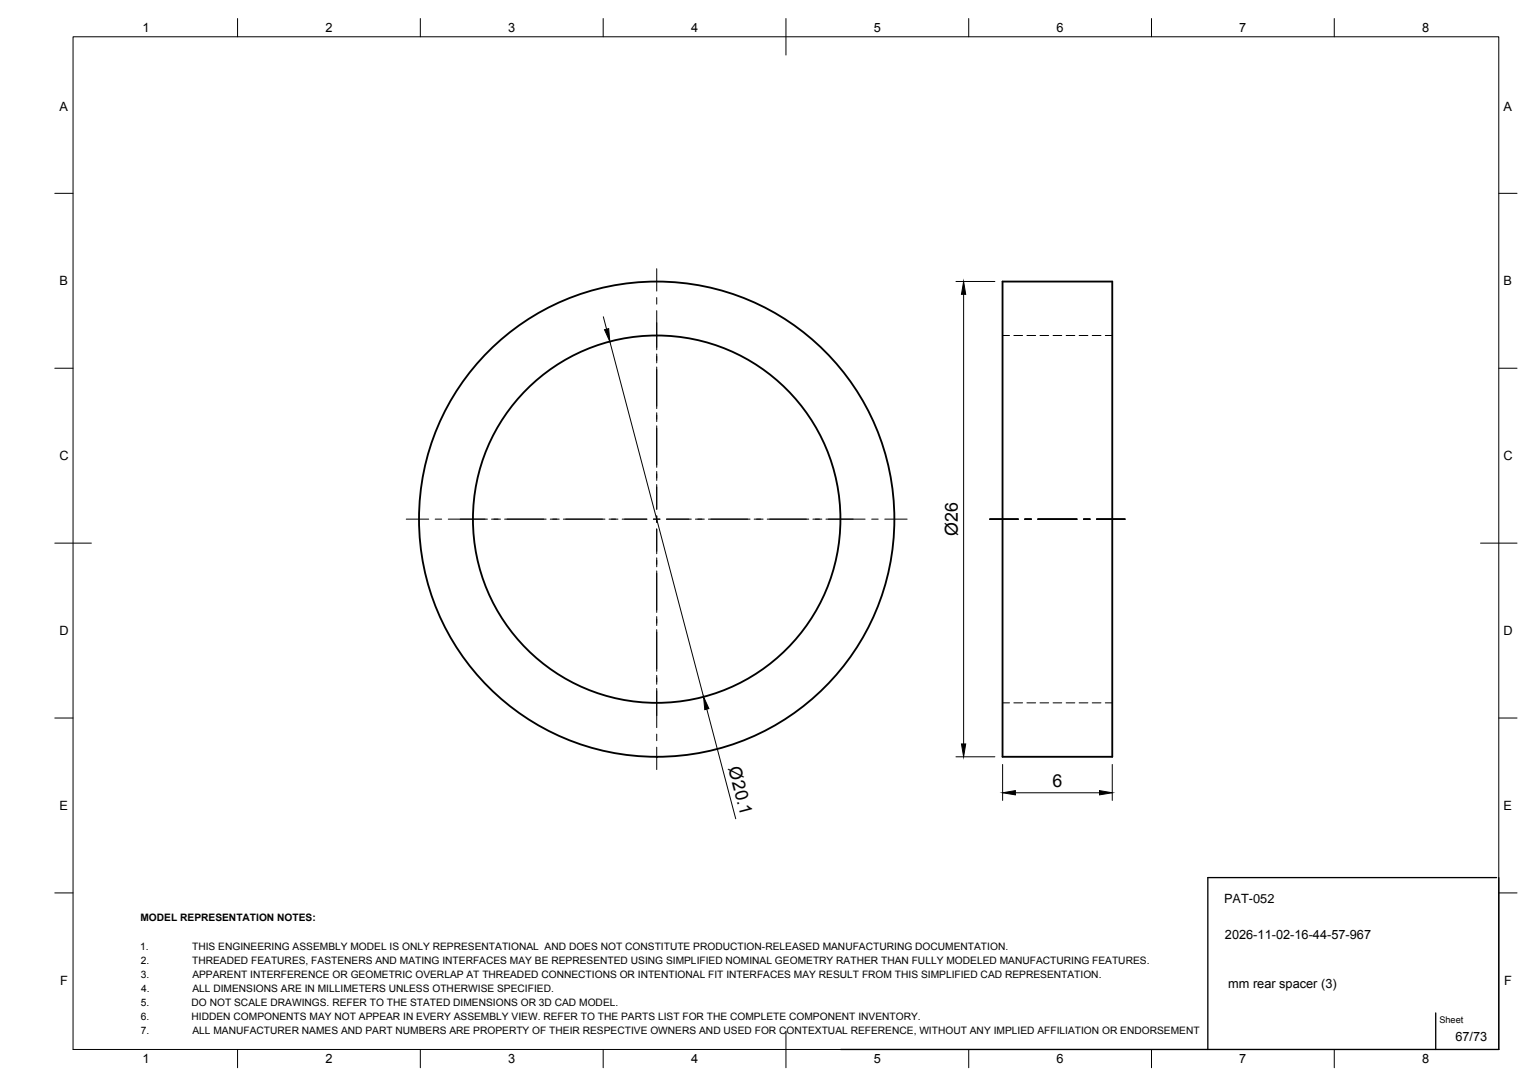
ISO-10303-21;
HEADER;
/* Generated by software containing ST-Developer
 * from STEP Tools, Inc. (www.steptools.com) 
 */

FILE_DESCRIPTION(
/* description */ ('Hand-crank gear train demonstrator'),
/* implementation_level */ '2;1');

FILE_NAME(
/* name */ 'mm rear spacer (3).step',
/* time_stamp */ '2026-10-28T03:22:13-07:00',
/* author */ (''),
/* organization */ (''),
/* preprocessor_version */ 'ST-DEVELOPER v20.2',
/* originating_system */ 'Autodesk Translation Framework v15.17.0.0',
/* authorisation */ '');

FILE_SCHEMA (('AUTOMOTIVE_DESIGN { 1 0 10303 214 3 1 1 }'));
ENDSEC;

DATA;
#10=MECHANICAL_DESIGN_GEOMETRIC_PRESENTATION_REPRESENTATION('',(#1257),#62758);
#1114=SHAPE_REPRESENTATION_RELATIONSHIP('SRR','None',#63092,#1178);
#1178=ADVANCED_BREP_SHAPE_REPRESENTATION('',(#1332),#62746);
#1257=STYLED_ITEM('',(#63476),#1332);
#1332=MANIFOLD_SOLID_BREP('Body1',#16441);
#1609=FACE_BOUND('',#4020,.T.);
#1610=FACE_BOUND('',#4022,.T.);
#2025=PLANE('',#18417);
#2026=PLANE('',#18418);
#2814=FACE_OUTER_BOUND('',#4017,.T.);
#2815=FACE_OUTER_BOUND('',#4018,.T.);
#2816=FACE_OUTER_BOUND('',#4019,.T.);
#2817=FACE_OUTER_BOUND('',#4021,.T.);
#4017=EDGE_LOOP('',(#13873,#13874,#13875,#13876));
#4018=EDGE_LOOP('',(#13877,#13878,#13879,#13880));
#4019=EDGE_LOOP('',(#13881));
#4020=EDGE_LOOP('',(#13882));
#4021=EDGE_LOOP('',(#13883));
#4022=EDGE_LOOP('',(#13884));
#5151=LINE('',#38498,#6283);
#5152=LINE('',#38504,#6284);
#6283=VECTOR('',#22206,1.005);
#6284=VECTOR('',#22213,1.3);
#7080=CIRCLE('',#18412,1.005);
#7081=CIRCLE('',#18413,1.005);
#7082=CIRCLE('',#18415,1.3);
#7083=CIRCLE('',#18416,1.3);
#8239=VERTEX_POINT('',#38495);
#8240=VERTEX_POINT('',#38497);
#8241=VERTEX_POINT('',#38501);
#8242=VERTEX_POINT('',#38503);
#10188=EDGE_CURVE('',#8239,#8239,#7080,.T.);
#10189=EDGE_CURVE('',#8239,#8240,#5151,.T.);
#10190=EDGE_CURVE('',#8240,#8240,#7081,.T.);
#10191=EDGE_CURVE('',#8241,#8241,#7082,.T.);
#10192=EDGE_CURVE('',#8241,#8242,#5152,.T.);
#10193=EDGE_CURVE('',#8242,#8242,#7083,.T.);
#13873=ORIENTED_EDGE('',*,*,#10188,.F.);
#13874=ORIENTED_EDGE('',*,*,#10189,.T.);
#13875=ORIENTED_EDGE('',*,*,#10190,.T.);
#13876=ORIENTED_EDGE('',*,*,#10189,.F.);
#13877=ORIENTED_EDGE('',*,*,#10191,.F.);
#13878=ORIENTED_EDGE('',*,*,#10192,.T.);
#13879=ORIENTED_EDGE('',*,*,#10193,.T.);
#13880=ORIENTED_EDGE('',*,*,#10192,.F.);
#13881=ORIENTED_EDGE('',*,*,#10191,.T.);
#13882=ORIENTED_EDGE('',*,*,#10188,.T.);
#13883=ORIENTED_EDGE('',*,*,#10193,.F.);
#13884=ORIENTED_EDGE('',*,*,#10190,.F.);
#15372=CYLINDRICAL_SURFACE('',#18411,1.005);
#15373=CYLINDRICAL_SURFACE('',#18414,1.3);
#16124=ADVANCED_FACE('',(#2814),#15372,.F.);
#16125=ADVANCED_FACE('',(#2815),#15373,.T.);
#16126=ADVANCED_FACE('',(#2816,#1609),#2025,.T.);
#16127=ADVANCED_FACE('',(#2817,#1610),#2026,.F.);
#16441=CLOSED_SHELL('',(#16124,#16125,#16126,#16127));
#18410=AXIS2_PLACEMENT_3D('',#38493,#22200,#22201);
#18411=AXIS2_PLACEMENT_3D('',#38494,#22202,#22203);
#18412=AXIS2_PLACEMENT_3D('',#38496,#22204,#22205);
#18413=AXIS2_PLACEMENT_3D('',#38499,#22207,#22208);
#18414=AXIS2_PLACEMENT_3D('',#38500,#22209,#22210);
#18415=AXIS2_PLACEMENT_3D('',#38502,#22211,#22212);
#18416=AXIS2_PLACEMENT_3D('',#38505,#22214,#22215);
#18417=AXIS2_PLACEMENT_3D('',#38506,#22216,#22217);
#18418=AXIS2_PLACEMENT_3D('',#38507,#22218,#22219);
#22200=DIRECTION('axis',(0.,0.,1.));
#22201=DIRECTION('refdir',(1.,0.,0.));
#22202=DIRECTION('center_axis',(0.,1.,0.));
#22203=DIRECTION('ref_axis',(1.,0.,0.));
#22204=DIRECTION('center_axis',(0.,-1.,0.));
#22205=DIRECTION('ref_axis',(1.,0.,0.));
#22206=DIRECTION('',(0.,-1.,0.));
#22207=DIRECTION('center_axis',(0.,-1.,0.));
#22208=DIRECTION('ref_axis',(1.,0.,0.));
#22209=DIRECTION('center_axis',(0.,1.,0.));
#22210=DIRECTION('ref_axis',(1.,0.,0.));
#22211=DIRECTION('center_axis',(0.,1.,0.));
#22212=DIRECTION('ref_axis',(1.,0.,0.));
#22213=DIRECTION('',(0.,-1.,0.));
#22214=DIRECTION('center_axis',(0.,1.,0.));
#22215=DIRECTION('ref_axis',(1.,0.,0.));
#22216=DIRECTION('center_axis',(0.,1.,0.));
#22217=DIRECTION('ref_axis',(1.,0.,0.));
#22218=DIRECTION('center_axis',(0.,1.,0.));
#22219=DIRECTION('ref_axis',(1.,0.,0.));
#38493=CARTESIAN_POINT('',(0.,0.,0.));
#38494=CARTESIAN_POINT('Origin',(18.,-2.8,9.));
#38495=CARTESIAN_POINT('',(16.995,-2.2,9.));
#38496=CARTESIAN_POINT('Origin',(18.,-2.2,9.));
#38497=CARTESIAN_POINT('',(16.995,-2.8,9.));
#38498=CARTESIAN_POINT('',(16.995,-2.8,9.));
#38499=CARTESIAN_POINT('Origin',(18.,-2.8,9.));
#38500=CARTESIAN_POINT('Origin',(18.,-2.8,9.));
#38501=CARTESIAN_POINT('',(16.7,-2.2,9.));
#38502=CARTESIAN_POINT('Origin',(18.,-2.2,9.));
#38503=CARTESIAN_POINT('',(16.7,-2.8,9.));
#38504=CARTESIAN_POINT('',(16.7,-2.8,9.));
#38505=CARTESIAN_POINT('Origin',(18.,-2.8,9.));
#38506=CARTESIAN_POINT('Origin',(18.,-2.2,9.));
#38507=CARTESIAN_POINT('Origin',(18.,-2.8,9.));
#62672=UNCERTAINTY_MEASURE_WITH_UNIT(LENGTH_MEASURE(0.001),#62759,
'DISTANCE_ACCURACY_VALUE',
'Maximum model space distance between geometric entities at asserted c
onnectivities');
#62684=UNCERTAINTY_MEASURE_WITH_UNIT(LENGTH_MEASURE(0.001),#62759,
'DISTANCE_ACCURACY_VALUE',
'Maximum model space distance between geometric entities at asserted c
onnectivities');
#62746=(
GEOMETRIC_REPRESENTATION_CONTEXT(3)
GLOBAL_UNCERTAINTY_ASSIGNED_CONTEXT((#62672))
GLOBAL_UNIT_ASSIGNED_CONTEXT((#62759,#62761,#62762))
REPRESENTATION_CONTEXT('','3D')
);
#62758=(
GEOMETRIC_REPRESENTATION_CONTEXT(3)
GLOBAL_UNCERTAINTY_ASSIGNED_CONTEXT((#62684))
GLOBAL_UNIT_ASSIGNED_CONTEXT((#62759,#62761,#62762))
REPRESENTATION_CONTEXT('','3D')
);
#62759=(
LENGTH_UNIT()
NAMED_UNIT(*)
SI_UNIT(.CENTI.,.METRE.)
);
#62761=(
NAMED_UNIT(*)
PLANE_ANGLE_UNIT()
SI_UNIT($,.RADIAN.)
);
#62762=(
NAMED_UNIT(*)
SI_UNIT($,.STERADIAN.)
SOLID_ANGLE_UNIT()
);
#62824=SHAPE_DEFINITION_REPRESENTATION(#62907,#63092);
#62907=PRODUCT_DEFINITION_SHAPE('',$,#63166);
#63092=SHAPE_REPRESENTATION('',(#18410),#62746);
#63104=PRODUCT_DEFINITION_CONTEXT('part definition',#63325,'design');
#63166=PRODUCT_DEFINITION('mm rear spacer (3)','mm rear spacer (3)',#63239,
#63104);
#63239=PRODUCT_DEFINITION_FORMATION('',$,#63388);
#63325=APPLICATION_CONTEXT(
'Core Data for Automotive Mechanical Design Process');
#63326=PRODUCT_CONTEXT('part definition',#63325,'mechanical');
#63388=PRODUCT('mm rear spacer (3)','mm rear spacer (3)','mm rear spacer (3)',
(#63326));
#63470=COLOUR_RGB('Off White',0.89,0.88,0.83);
#63471=FILL_AREA_STYLE_COLOUR('',#63470);
#63472=FILL_AREA_STYLE('',(#63471));
#63473=SURFACE_STYLE_FILL_AREA(#63472);
#63474=SURFACE_SIDE_STYLE('',(#63473));
#63475=SURFACE_STYLE_USAGE(.BOTH.,#63474);
#63476=PRESENTATION_STYLE_ASSIGNMENT((#63475));
ENDSEC;
END-ISO-10303-21;
